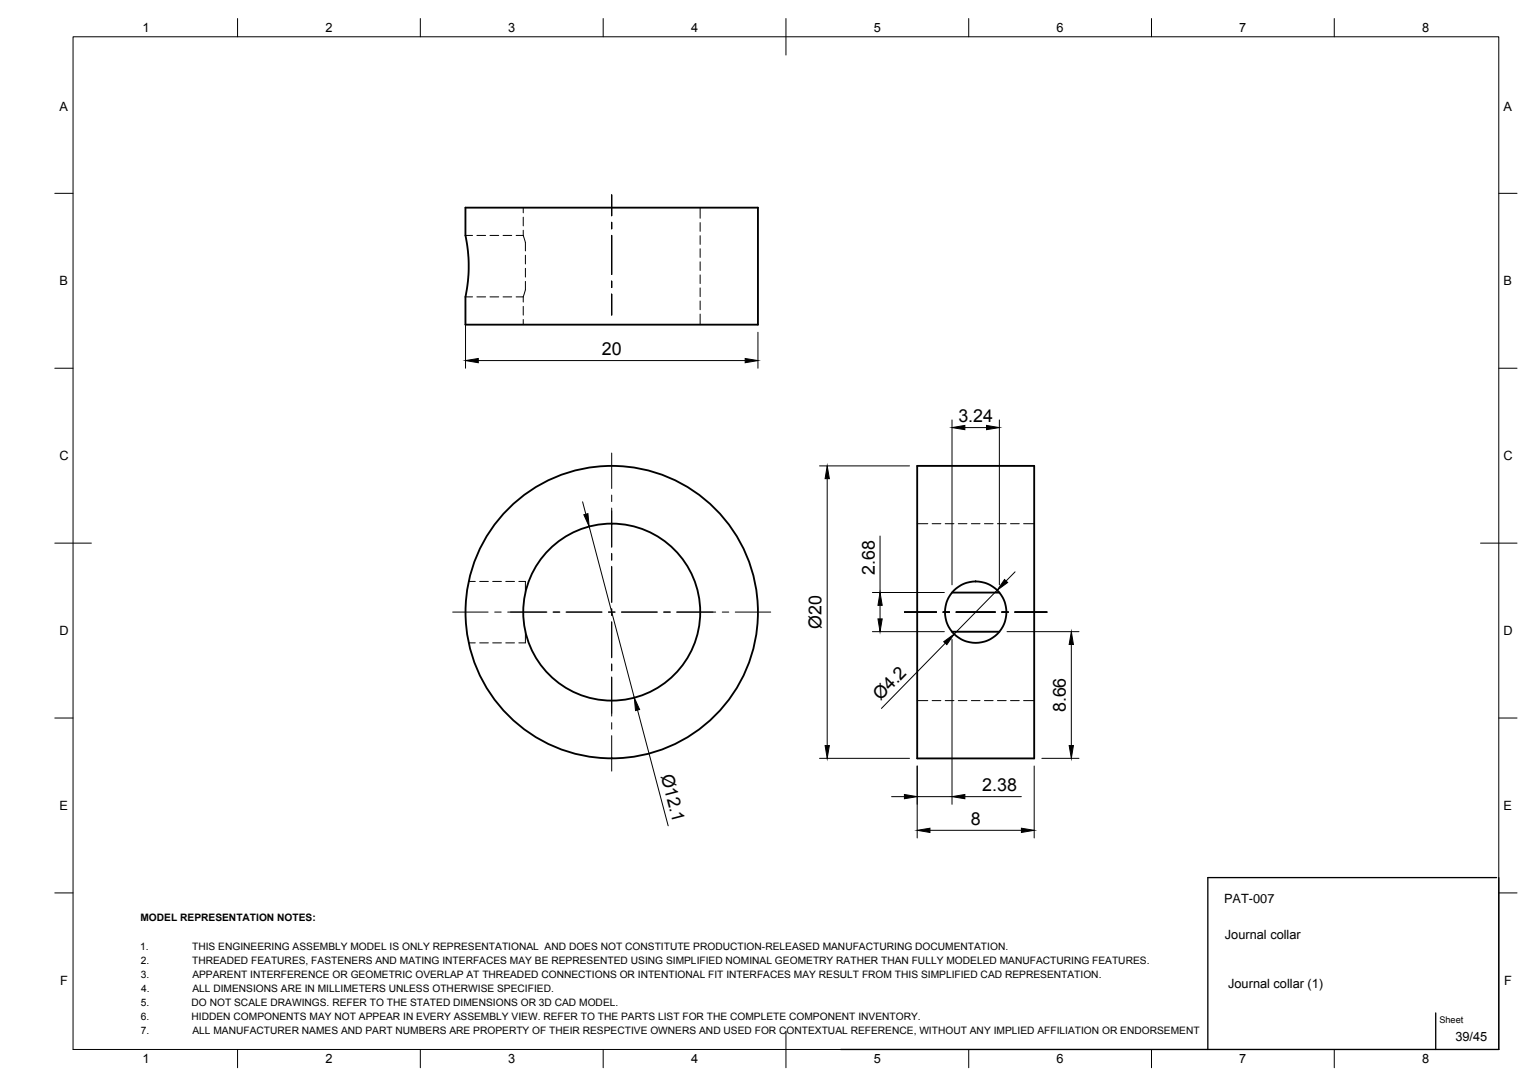
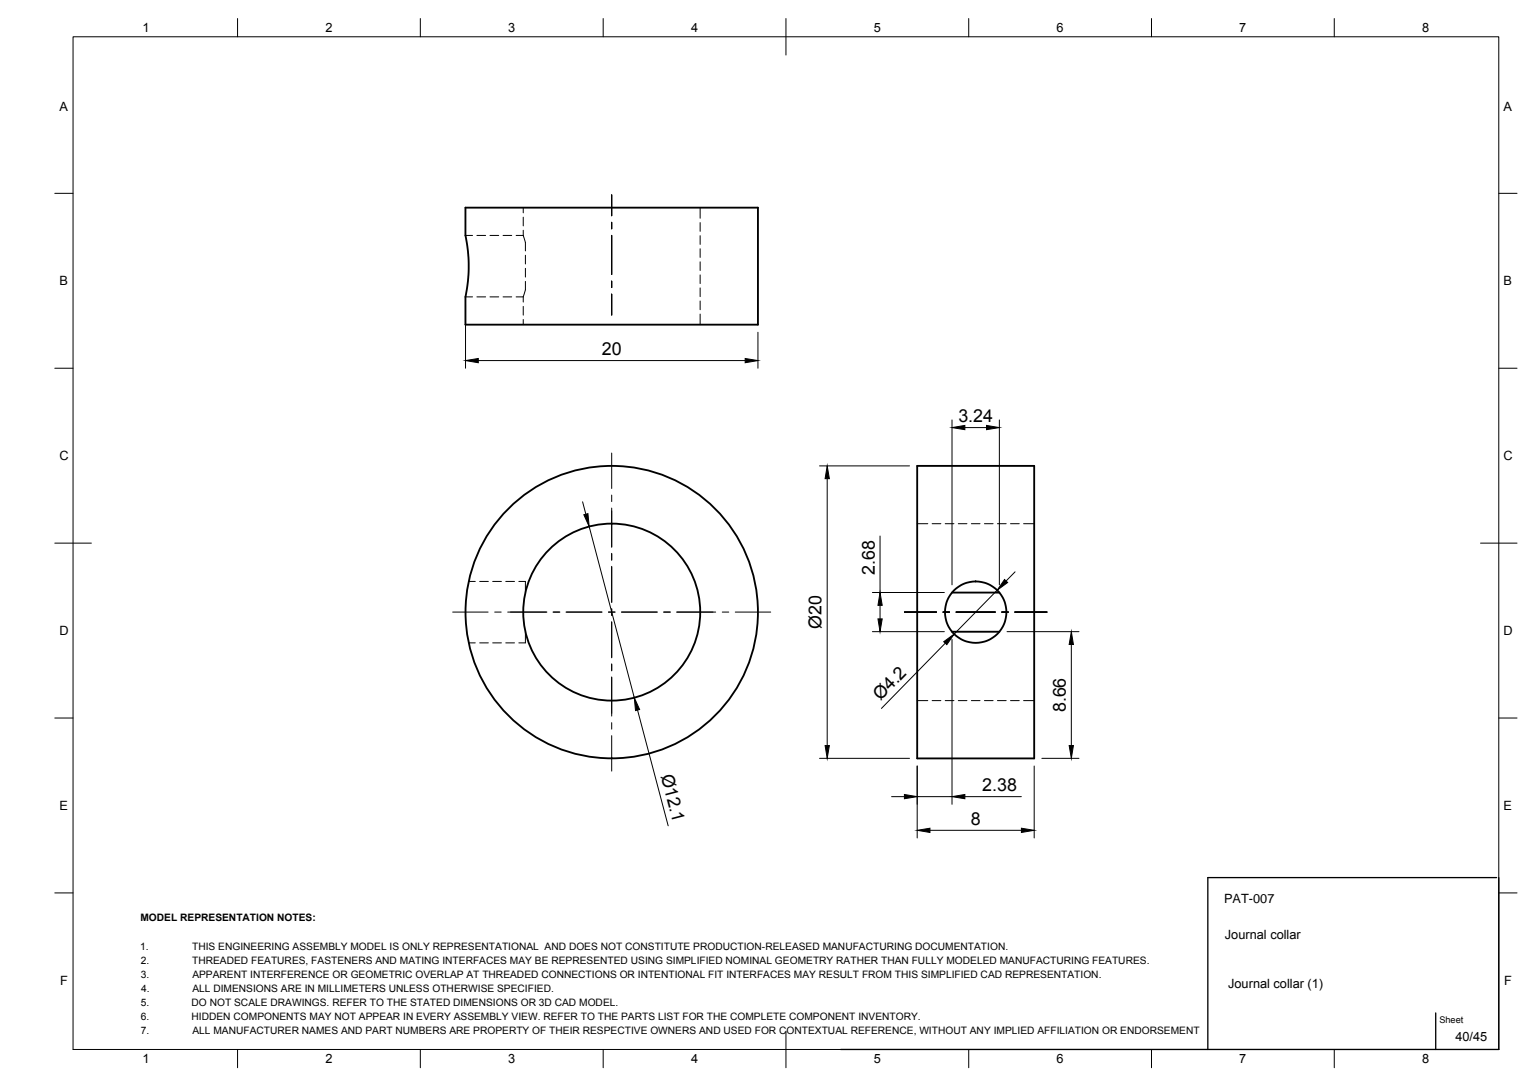
ISO-10303-21;
HEADER;
/* Generated by software containing ST-Developer
 * from STEP Tools, Inc. (www.steptools.com) 
 */

FILE_DESCRIPTION(
/* description */ ('Bearing friction torque test rig'),
/* implementation_level */ '2;1');

FILE_NAME(
/* name */ 'Journal collar.step',
/* time_stamp */ '2026-10-28T03:24:04-07:00',
/* author */ (''),
/* organization */ (''),
/* preprocessor_version */ 'ST-DEVELOPER v20.2',
/* originating_system */ 'Autodesk Translation Framework v15.17.0.0',
/* authorisation */ '');

FILE_SCHEMA (('AUTOMOTIVE_DESIGN { 1 0 10303 214 3 1 1 }'));
ENDSEC;

DATA;
#10=MECHANICAL_DESIGN_GEOMETRIC_PRESENTATION_REPRESENTATION('',(#585),#14822);
#375=B_SPLINE_CURVE_WITH_KNOTS('',3,(#14158,#14159,#14160,#14161,#14162,
#14163,#14164,#14165,#14166,#14167),.UNSPECIFIED.,.F.,.F.,(4,2,2,2,4),(0.818088904349174,
0.878131747417166,0.957937926194037,1.03774410497091,1.0977869480389),
 .UNSPECIFIED.);
#376=B_SPLINE_CURVE_WITH_KNOTS('',3,(#14173,#14174,#14175,#14176,#14177,
#14178,#14179,#14180,#14181,#14182,#14183,#14184,#14185,#14186,#14187,#14188,
#14189,#14190),.UNSPECIFIED.,.F.,.F.,(4,2,2,2,2,2,2,2,4),(0.,0.0793616477694787,
0.158723295538957,0.238079516586307,0.317435737633657,0.396791958681006,
0.476148179728356,0.555509827497835,0.634871475267313),.UNSPECIFIED.);
#377=B_SPLINE_CURVE_WITH_KNOTS('',3,(#14191,#14192,#14193,#14194,#14195,
#14196,#14197,#14198,#14199,#14200,#14201,#14202,#14203,#14204,#14205,#14206,
#14207,#14208),.UNSPECIFIED.,.F.,.F.,(4,2,2,2,2,2,2,2,4),(0.634871475267313,
0.714233123036792,0.793594770806271,0.87295099185362,0.95230721290097,1.03166343394832,
1.11101965499567,1.19038130276515,1.26974295053463),.UNSPECIFIED.);
#378=B_SPLINE_CURVE_WITH_KNOTS('',3,(#14211,#14212,#14213,#14214,#14215,
#14216,#14217,#14218,#14219,#14220),.UNSPECIFIED.,.F.,.F.,(4,2,2,2,4),(0.179463620219816,
0.239506463287808,0.319312642064679,0.39911882084155,0.459161663909542),
 .UNSPECIFIED.);
#492=SHAPE_REPRESENTATION_RELATIONSHIP('SRR','None',#15034,#531);
#531=ADVANCED_BREP_SHAPE_REPRESENTATION('',(#636),#14814);
#585=STYLED_ITEM('',(#15277),#636);
#636=MANIFOLD_SOLID_BREP('Body1',#7704);
#840=FACE_BOUND('',#2128,.T.);
#841=FACE_BOUND('',#2130,.T.);
#842=FACE_BOUND('',#2132,.T.);
#843=FACE_BOUND('',#2134,.T.);
#1065=PLANE('',#9024);
#1066=PLANE('',#9029);
#1067=PLANE('',#9036);
#1068=PLANE('',#9037);
#1483=FACE_OUTER_BOUND('',#2124,.T.);
#1484=FACE_OUTER_BOUND('',#2125,.T.);
#1485=FACE_OUTER_BOUND('',#2126,.T.);
#1486=FACE_OUTER_BOUND('',#2127,.T.);
#1487=FACE_OUTER_BOUND('',#2129,.T.);
#1488=FACE_OUTER_BOUND('',#2131,.T.);
#1489=FACE_OUTER_BOUND('',#2133,.T.);
#2124=EDGE_LOOP('',(#6780,#6781));
#2125=EDGE_LOOP('',(#6782,#6783,#6784,#6785,#6786,#6787,#6788,#6789,#6790));
#2126=EDGE_LOOP('',(#6791,#6792,#6793));
#2127=EDGE_LOOP('',(#6794,#6795,#6796,#6797));
#2128=EDGE_LOOP('',(#6798,#6799,#6800,#6801));
#2129=EDGE_LOOP('',(#6802,#6803,#6804,#6805));
#2130=EDGE_LOOP('',(#6806,#6807));
#2131=EDGE_LOOP('',(#6808));
#2132=EDGE_LOOP('',(#6809));
#2133=EDGE_LOOP('',(#6810));
#2134=EDGE_LOOP('',(#6811));
#2608=LINE('',#14154,#3052);
#2609=LINE('',#14171,#3053);
#2610=LINE('',#14222,#3054);
#2611=LINE('',#14227,#3055);
#2612=LINE('',#14233,#3056);
#3052=VECTOR('',#11321,1.);
#3053=VECTOR('',#11328,0.21);
#3054=VECTOR('',#11333,1.);
#3055=VECTOR('',#11338,0.605);
#3056=VECTOR('',#11345,1.);
#3496=CIRCLE('',#9025,0.21);
#3497=CIRCLE('',#9027,0.21);
#3498=CIRCLE('',#9028,0.21);
#3499=CIRCLE('',#9031,0.605);
#3500=CIRCLE('',#9032,0.605);
#3501=CIRCLE('',#9034,1.);
#3502=CIRCLE('',#9035,1.);
#4111=VERTEX_POINT('',#14152);
#4112=VERTEX_POINT('',#14153);
#4113=VERTEX_POINT('',#14157);
#4114=VERTEX_POINT('',#14168);
#4115=VERTEX_POINT('',#14170);
#4116=VERTEX_POINT('',#14172);
#4117=VERTEX_POINT('',#14209);
#4118=VERTEX_POINT('',#14224);
#4119=VERTEX_POINT('',#14226);
#4120=VERTEX_POINT('',#14230);
#4121=VERTEX_POINT('',#14232);
#5016=EDGE_CURVE('',#4111,#4112,#2608,.T.);
#5017=EDGE_CURVE('',#4111,#4112,#3496,.T.);
#5018=EDGE_CURVE('',#4113,#4111,#375,.T.);
#5019=EDGE_CURVE('',#4114,#4113,#3497,.T.);
#5020=EDGE_CURVE('',#4114,#4115,#2609,.T.);
#5021=EDGE_CURVE('',#4116,#4115,#376,.T.);
#5022=EDGE_CURVE('',#4115,#4116,#377,.T.);
#5023=EDGE_CURVE('',#4117,#4114,#3498,.T.);
#5024=EDGE_CURVE('',#4112,#4117,#378,.T.);
#5025=EDGE_CURVE('',#4117,#4113,#2610,.T.);
#5026=EDGE_CURVE('',#4118,#4118,#3499,.T.);
#5027=EDGE_CURVE('',#4118,#4119,#2611,.T.);
#5028=EDGE_CURVE('',#4119,#4119,#3500,.T.);
#5029=EDGE_CURVE('',#4120,#4120,#3501,.T.);
#5030=EDGE_CURVE('',#4120,#4121,#2612,.T.);
#5031=EDGE_CURVE('',#4121,#4121,#3502,.T.);
#6780=ORIENTED_EDGE('',*,*,#5016,.F.);
#6781=ORIENTED_EDGE('',*,*,#5017,.T.);
#6782=ORIENTED_EDGE('',*,*,#5018,.F.);
#6783=ORIENTED_EDGE('',*,*,#5019,.F.);
#6784=ORIENTED_EDGE('',*,*,#5020,.T.);
#6785=ORIENTED_EDGE('',*,*,#5021,.F.);
#6786=ORIENTED_EDGE('',*,*,#5022,.F.);
#6787=ORIENTED_EDGE('',*,*,#5020,.F.);
#6788=ORIENTED_EDGE('',*,*,#5023,.F.);
#6789=ORIENTED_EDGE('',*,*,#5024,.F.);
#6790=ORIENTED_EDGE('',*,*,#5017,.F.);
#6791=ORIENTED_EDGE('',*,*,#5025,.F.);
#6792=ORIENTED_EDGE('',*,*,#5023,.T.);
#6793=ORIENTED_EDGE('',*,*,#5019,.T.);
#6794=ORIENTED_EDGE('',*,*,#5026,.F.);
#6795=ORIENTED_EDGE('',*,*,#5027,.T.);
#6796=ORIENTED_EDGE('',*,*,#5028,.T.);
#6797=ORIENTED_EDGE('',*,*,#5027,.F.);
#6798=ORIENTED_EDGE('',*,*,#5024,.T.);
#6799=ORIENTED_EDGE('',*,*,#5025,.T.);
#6800=ORIENTED_EDGE('',*,*,#5018,.T.);
#6801=ORIENTED_EDGE('',*,*,#5016,.T.);
#6802=ORIENTED_EDGE('',*,*,#5029,.F.);
#6803=ORIENTED_EDGE('',*,*,#5030,.T.);
#6804=ORIENTED_EDGE('',*,*,#5031,.T.);
#6805=ORIENTED_EDGE('',*,*,#5030,.F.);
#6806=ORIENTED_EDGE('',*,*,#5021,.T.);
#6807=ORIENTED_EDGE('',*,*,#5022,.T.);
#6808=ORIENTED_EDGE('',*,*,#5029,.T.);
#6809=ORIENTED_EDGE('',*,*,#5026,.T.);
#6810=ORIENTED_EDGE('',*,*,#5031,.F.);
#6811=ORIENTED_EDGE('',*,*,#5028,.F.);
#7185=CYLINDRICAL_SURFACE('',#9026,0.21);
#7186=CYLINDRICAL_SURFACE('',#9030,0.605);
#7187=CYLINDRICAL_SURFACE('',#9033,1.);
#7594=ADVANCED_FACE('',(#1483),#1065,.T.);
#7595=ADVANCED_FACE('',(#1484),#7185,.F.);
#7596=ADVANCED_FACE('',(#1485),#1066,.T.);
#7597=ADVANCED_FACE('',(#1486,#840),#7186,.F.);
#7598=ADVANCED_FACE('',(#1487,#841),#7187,.T.);
#7599=ADVANCED_FACE('',(#1488,#842),#1067,.T.);
#7600=ADVANCED_FACE('',(#1489,#843),#1068,.F.);
#7704=CLOSED_SHELL('',(#7594,#7595,#7596,#7597,#7598,#7599,#7600));
#9023=AXIS2_PLACEMENT_3D('',#14150,#11317,#11318);
#9024=AXIS2_PLACEMENT_3D('',#14151,#11319,#11320);
#9025=AXIS2_PLACEMENT_3D('',#14155,#11322,#11323);
#9026=AXIS2_PLACEMENT_3D('',#14156,#11324,#11325);
#9027=AXIS2_PLACEMENT_3D('',#14169,#11326,#11327);
#9028=AXIS2_PLACEMENT_3D('',#14210,#11329,#11330);
#9029=AXIS2_PLACEMENT_3D('',#14221,#11331,#11332);
#9030=AXIS2_PLACEMENT_3D('',#14223,#11334,#11335);
#9031=AXIS2_PLACEMENT_3D('',#14225,#11336,#11337);
#9032=AXIS2_PLACEMENT_3D('',#14228,#11339,#11340);
#9033=AXIS2_PLACEMENT_3D('',#14229,#11341,#11342);
#9034=AXIS2_PLACEMENT_3D('',#14231,#11343,#11344);
#9035=AXIS2_PLACEMENT_3D('',#14234,#11346,#11347);
#9036=AXIS2_PLACEMENT_3D('',#14235,#11348,#11349);
#9037=AXIS2_PLACEMENT_3D('',#14236,#11350,#11351);
#11317=DIRECTION('axis',(0.,0.,1.));
#11318=DIRECTION('refdir',(1.,0.,0.));
#11319=DIRECTION('center_axis',(0.,0.,1.));
#11320=DIRECTION('ref_axis',(1.,0.,0.));
#11321=DIRECTION('',(0.,1.,0.));
#11322=DIRECTION('center_axis',(0.,0.,1.));
#11323=DIRECTION('ref_axis',(1.,0.,0.));
#11324=DIRECTION('center_axis',(0.,0.,1.));
#11325=DIRECTION('ref_axis',(1.,0.,0.));
#11326=DIRECTION('center_axis',(0.,0.,1.));
#11327=DIRECTION('ref_axis',(1.,0.,0.));
#11328=DIRECTION('',(0.,0.,1.));
#11329=DIRECTION('center_axis',(0.,0.,1.));
#11330=DIRECTION('ref_axis',(1.,0.,0.));
#11331=DIRECTION('center_axis',(0.,0.,1.));
#11332=DIRECTION('ref_axis',(1.,0.,0.));
#11333=DIRECTION('',(0.,-1.,0.));
#11334=DIRECTION('center_axis',(0.,1.,0.));
#11335=DIRECTION('ref_axis',(1.,0.,0.));
#11336=DIRECTION('center_axis',(0.,-1.,0.));
#11337=DIRECTION('ref_axis',(1.,0.,0.));
#11338=DIRECTION('',(0.,-1.,0.));
#11339=DIRECTION('center_axis',(0.,-1.,0.));
#11340=DIRECTION('ref_axis',(1.,0.,0.));
#11341=DIRECTION('center_axis',(0.,1.,0.));
#11342=DIRECTION('ref_axis',(1.,0.,0.));
#11343=DIRECTION('center_axis',(0.,1.,0.));
#11344=DIRECTION('ref_axis',(1.,0.,0.));
#11345=DIRECTION('',(0.,-1.,0.));
#11346=DIRECTION('center_axis',(0.,1.,0.));
#11347=DIRECTION('ref_axis',(1.,0.,0.));
#11348=DIRECTION('center_axis',(0.,1.,0.));
#11349=DIRECTION('ref_axis',(1.,0.,0.));
#11350=DIRECTION('center_axis',(0.,1.,0.));
#11351=DIRECTION('ref_axis',(1.,0.,0.));
#14150=CARTESIAN_POINT('',(0.,0.,0.));
#14151=CARTESIAN_POINT('Origin',(0.,-8.6,7.59));
#14152=CARTESIAN_POINT('',(0.133884278389956,-8.76178689687364,7.59));
#14153=CARTESIAN_POINT('',(0.133884278389956,-8.43821310312636,7.59));
#14154=CARTESIAN_POINT('',(0.133884278389956,-9.,7.59));
#14155=CARTESIAN_POINT('Origin',(0.,-8.6,7.59));
#14156=CARTESIAN_POINT('Origin',(0.,-8.6,7.59));
#14157=CARTESIAN_POINT('',(-0.133884278389956,-8.76178689687364,7.59));
#14158=CARTESIAN_POINT('Ctrl Pts',(-0.133884278389955,-8.76178689687364,
7.59));
#14159=CARTESIAN_POINT('Ctrl Pts',(-0.118254395260799,-8.77472116821763,
7.59354677224418));
#14160=CARTESIAN_POINT('Ctrl Pts',(-0.100109787682298,-8.78579931658744,
7.59698224789957));
#14161=CARTESIAN_POINT('Ctrl Pts',(-0.054829872132519,-8.80463856105443,
7.6030741628997));
#14162=CARTESIAN_POINT('Ctrl Pts',(-0.0266020595922903,-8.81,7.605));
#14163=CARTESIAN_POINT('Ctrl Pts',(0.0266020595922903,-8.81,7.605));
#14164=CARTESIAN_POINT('Ctrl Pts',(0.0548298721325189,-8.80463856105443,
7.6030741628997));
#14165=CARTESIAN_POINT('Ctrl Pts',(0.100109787682298,-8.78579931658744,
7.59698224789957));
#14166=CARTESIAN_POINT('Ctrl Pts',(0.118254395260801,-8.77472116821763,
7.59354677224418));
#14167=CARTESIAN_POINT('Ctrl Pts',(0.133884278389955,-8.76178689687364,
7.59));
#14168=CARTESIAN_POINT('',(-0.21,-8.6,7.59));
#14169=CARTESIAN_POINT('Origin',(0.,-8.6,7.59));
#14170=CARTESIAN_POINT('',(-0.21,-8.6,7.97770138590472));
#14171=CARTESIAN_POINT('',(-0.21,-8.6,7.59));
#14172=CARTESIAN_POINT('',(0.21,-8.6,7.97770138590472));
#14173=CARTESIAN_POINT('Ctrl Pts',(0.21,-8.6,7.97770138590472));
#14174=CARTESIAN_POINT('Ctrl Pts',(0.21,-8.62645388258982,7.97770138590472));
#14175=CARTESIAN_POINT('Ctrl Pts',(0.204697017125528,-8.65461525830868,
7.97888646613217));
#14176=CARTESIAN_POINT('Ctrl Pts',(0.183241751515529,-8.70633042130174,
7.98312869991148));
#14177=CARTESIAN_POINT('Ctrl Pts',(0.167093586802906,-8.72989126129544,
7.98612044796649));
#14178=CARTESIAN_POINT('Ctrl Pts',(0.129892533236543,-8.76709231486181,
7.99170645156379));
#14179=CARTESIAN_POINT('Ctrl Pts',(0.106331154992714,-8.78324147510569,
7.99466914446598));
#14180=CARTESIAN_POINT('Ctrl Pts',(0.0546141143983522,-8.80469746372443,
7.99884449237241));
#14181=CARTESIAN_POINT('Ctrl Pts',(0.0264520736824499,-8.81,8.));
#14182=CARTESIAN_POINT('Ctrl Pts',(-0.0264520736824498,-8.81,8.));
#14183=CARTESIAN_POINT('Ctrl Pts',(-0.0546141143983521,-8.80469746372443,
7.99884449237241));
#14184=CARTESIAN_POINT('Ctrl Pts',(-0.106331154992714,-8.78324147510569,
7.99466914446598));
#14185=CARTESIAN_POINT('Ctrl Pts',(-0.129892533236543,-8.76709231486181,
7.99170645156379));
#14186=CARTESIAN_POINT('Ctrl Pts',(-0.167093586802906,-8.72989126129544,
7.98612044796649));
#14187=CARTESIAN_POINT('Ctrl Pts',(-0.183241751515529,-8.70633042130174,
7.98312869991148));
#14188=CARTESIAN_POINT('Ctrl Pts',(-0.204697017125528,-8.65461525830868,
7.97888646613217));
#14189=CARTESIAN_POINT('Ctrl Pts',(-0.21,-8.62645388258982,7.97770138590472));
#14190=CARTESIAN_POINT('Ctrl Pts',(-0.21,-8.6,7.97770138590472));
#14191=CARTESIAN_POINT('Ctrl Pts',(-0.21,-8.6,7.97770138590472));
#14192=CARTESIAN_POINT('Ctrl Pts',(-0.21,-8.57354611741017,7.97770138590472));
#14193=CARTESIAN_POINT('Ctrl Pts',(-0.204697017125528,-8.54538474169131,
7.97888646613217));
#14194=CARTESIAN_POINT('Ctrl Pts',(-0.183241751515529,-8.49366957869826,
7.98312869991148));
#14195=CARTESIAN_POINT('Ctrl Pts',(-0.167093586802906,-8.47010873870456,
7.98612044796649));
#14196=CARTESIAN_POINT('Ctrl Pts',(-0.129892533236543,-8.43290768513819,
7.99170645156379));
#14197=CARTESIAN_POINT('Ctrl Pts',(-0.106331154992714,-8.41675852489431,
7.99466914446598));
#14198=CARTESIAN_POINT('Ctrl Pts',(-0.0546141143983522,-8.39530253627557,
7.99884449237241));
#14199=CARTESIAN_POINT('Ctrl Pts',(-0.0264520736824499,-8.39,8.));
#14200=CARTESIAN_POINT('Ctrl Pts',(0.0264520736824499,-8.39,8.));
#14201=CARTESIAN_POINT('Ctrl Pts',(0.0546141143983517,-8.39530253627557,
7.99884449237241));
#14202=CARTESIAN_POINT('Ctrl Pts',(0.106331154992713,-8.41675852489431,
7.99466914446598));
#14203=CARTESIAN_POINT('Ctrl Pts',(0.129892533236543,-8.43290768513819,
7.99170645156379));
#14204=CARTESIAN_POINT('Ctrl Pts',(0.167093586802906,-8.47010873870456,
7.98612044796649));
#14205=CARTESIAN_POINT('Ctrl Pts',(0.183241751515529,-8.49366957869826,
7.98312869991148));
#14206=CARTESIAN_POINT('Ctrl Pts',(0.204697017125528,-8.54538474169131,
7.97888646613217));
#14207=CARTESIAN_POINT('Ctrl Pts',(0.21,-8.57354611741017,7.97770138590472));
#14208=CARTESIAN_POINT('Ctrl Pts',(0.21,-8.6,7.97770138590472));
#14209=CARTESIAN_POINT('',(-0.133884278389956,-8.43821310312636,7.59));
#14210=CARTESIAN_POINT('Origin',(0.,-8.6,7.59));
#14211=CARTESIAN_POINT('Ctrl Pts',(0.133884278389955,-8.43821310312636,
7.59));
#14212=CARTESIAN_POINT('Ctrl Pts',(0.118254395260801,-8.42527883178237,
7.59354677224418));
#14213=CARTESIAN_POINT('Ctrl Pts',(0.100109787682299,-8.41420068341256,
7.59698224789957));
#14214=CARTESIAN_POINT('Ctrl Pts',(0.054829872132519,-8.39536143894557,
7.6030741628997));
#14215=CARTESIAN_POINT('Ctrl Pts',(0.0266020595922903,-8.39,7.605));
#14216=CARTESIAN_POINT('Ctrl Pts',(-0.0266020595922903,-8.39,7.605));
#14217=CARTESIAN_POINT('Ctrl Pts',(-0.0548298721325189,-8.39536143894557,
7.6030741628997));
#14218=CARTESIAN_POINT('Ctrl Pts',(-0.100109787682299,-8.41420068341256,
7.59698224789957));
#14219=CARTESIAN_POINT('Ctrl Pts',(-0.118254395260801,-8.42527883178237,
7.59354677224418));
#14220=CARTESIAN_POINT('Ctrl Pts',(-0.133884278389955,-8.43821310312636,
7.59));
#14221=CARTESIAN_POINT('Origin',(0.,-8.6,7.59));
#14222=CARTESIAN_POINT('',(-0.133884278389956,-9.,7.59));
#14223=CARTESIAN_POINT('Origin',(0.,-9.,7.));
#14224=CARTESIAN_POINT('',(-0.605,-8.2,7.));
#14225=CARTESIAN_POINT('Origin',(0.,-8.2,7.));
#14226=CARTESIAN_POINT('',(-0.605,-9.,7.));
#14227=CARTESIAN_POINT('',(-0.605,-9.,7.));
#14228=CARTESIAN_POINT('Origin',(0.,-9.,7.));
#14229=CARTESIAN_POINT('Origin',(0.,-9.,7.));
#14230=CARTESIAN_POINT('',(-1.,-8.2,7.));
#14231=CARTESIAN_POINT('Origin',(0.,-8.2,7.));
#14232=CARTESIAN_POINT('',(-1.,-9.,7.));
#14233=CARTESIAN_POINT('',(-1.,-9.,7.));
#14234=CARTESIAN_POINT('Origin',(0.,-9.,7.));
#14235=CARTESIAN_POINT('Origin',(0.,-8.2,7.));
#14236=CARTESIAN_POINT('Origin',(0.,-9.,7.));
#14769=UNCERTAINTY_MEASURE_WITH_UNIT(LENGTH_MEASURE(0.001),#14823,
'DISTANCE_ACCURACY_VALUE',
'Maximum model space distance between geometric entities at asserted c
onnectivities');
#14777=UNCERTAINTY_MEASURE_WITH_UNIT(LENGTH_MEASURE(0.001),#14823,
'DISTANCE_ACCURACY_VALUE',
'Maximum model space distance between geometric entities at asserted c
onnectivities');
#14814=(
GEOMETRIC_REPRESENTATION_CONTEXT(3)
GLOBAL_UNCERTAINTY_ASSIGNED_CONTEXT((#14769))
GLOBAL_UNIT_ASSIGNED_CONTEXT((#14823,#14825,#14826))
REPRESENTATION_CONTEXT('','3D')
);
#14822=(
GEOMETRIC_REPRESENTATION_CONTEXT(3)
GLOBAL_UNCERTAINTY_ASSIGNED_CONTEXT((#14777))
GLOBAL_UNIT_ASSIGNED_CONTEXT((#14823,#14825,#14826))
REPRESENTATION_CONTEXT('','3D')
);
#14823=(
LENGTH_UNIT()
NAMED_UNIT(*)
SI_UNIT(.CENTI.,.METRE.)
);
#14825=(
NAMED_UNIT(*)
PLANE_ANGLE_UNIT()
SI_UNIT($,.RADIAN.)
);
#14826=(
NAMED_UNIT(*)
SI_UNIT($,.STERADIAN.)
SOLID_ANGLE_UNIT()
);
#14863=SHAPE_DEFINITION_REPRESENTATION(#14973,#15034);
#14973=PRODUCT_DEFINITION_SHAPE('',$,#15079);
#15034=SHAPE_REPRESENTATION('',(#9023),#14814);
#15042=PRODUCT_DEFINITION_CONTEXT('part definition',#15176,'design');
#15079=PRODUCT_DEFINITION('Journal collar','Journal collar',#15123,#15042);
#15123=PRODUCT_DEFINITION_FORMATION('',$,#15214);
#15176=APPLICATION_CONTEXT(
'Core Data for Automotive Mechanical Design Process');
#15177=PRODUCT_CONTEXT('part definition',#15176,'mechanical');
#15214=PRODUCT('Journal collar','Journal collar','Journal collar',(#15177));
#15271=COLOUR_RGB('Sky Blue',0.24,0.69,0.87);
#15272=FILL_AREA_STYLE_COLOUR('',#15271);
#15273=FILL_AREA_STYLE('',(#15272));
#15274=SURFACE_STYLE_FILL_AREA(#15273);
#15275=SURFACE_SIDE_STYLE('',(#15274));
#15276=SURFACE_STYLE_USAGE(.BOTH.,#15275);
#15277=PRESENTATION_STYLE_ASSIGNMENT((#15276));
ENDSEC;
END-ISO-10303-21;
